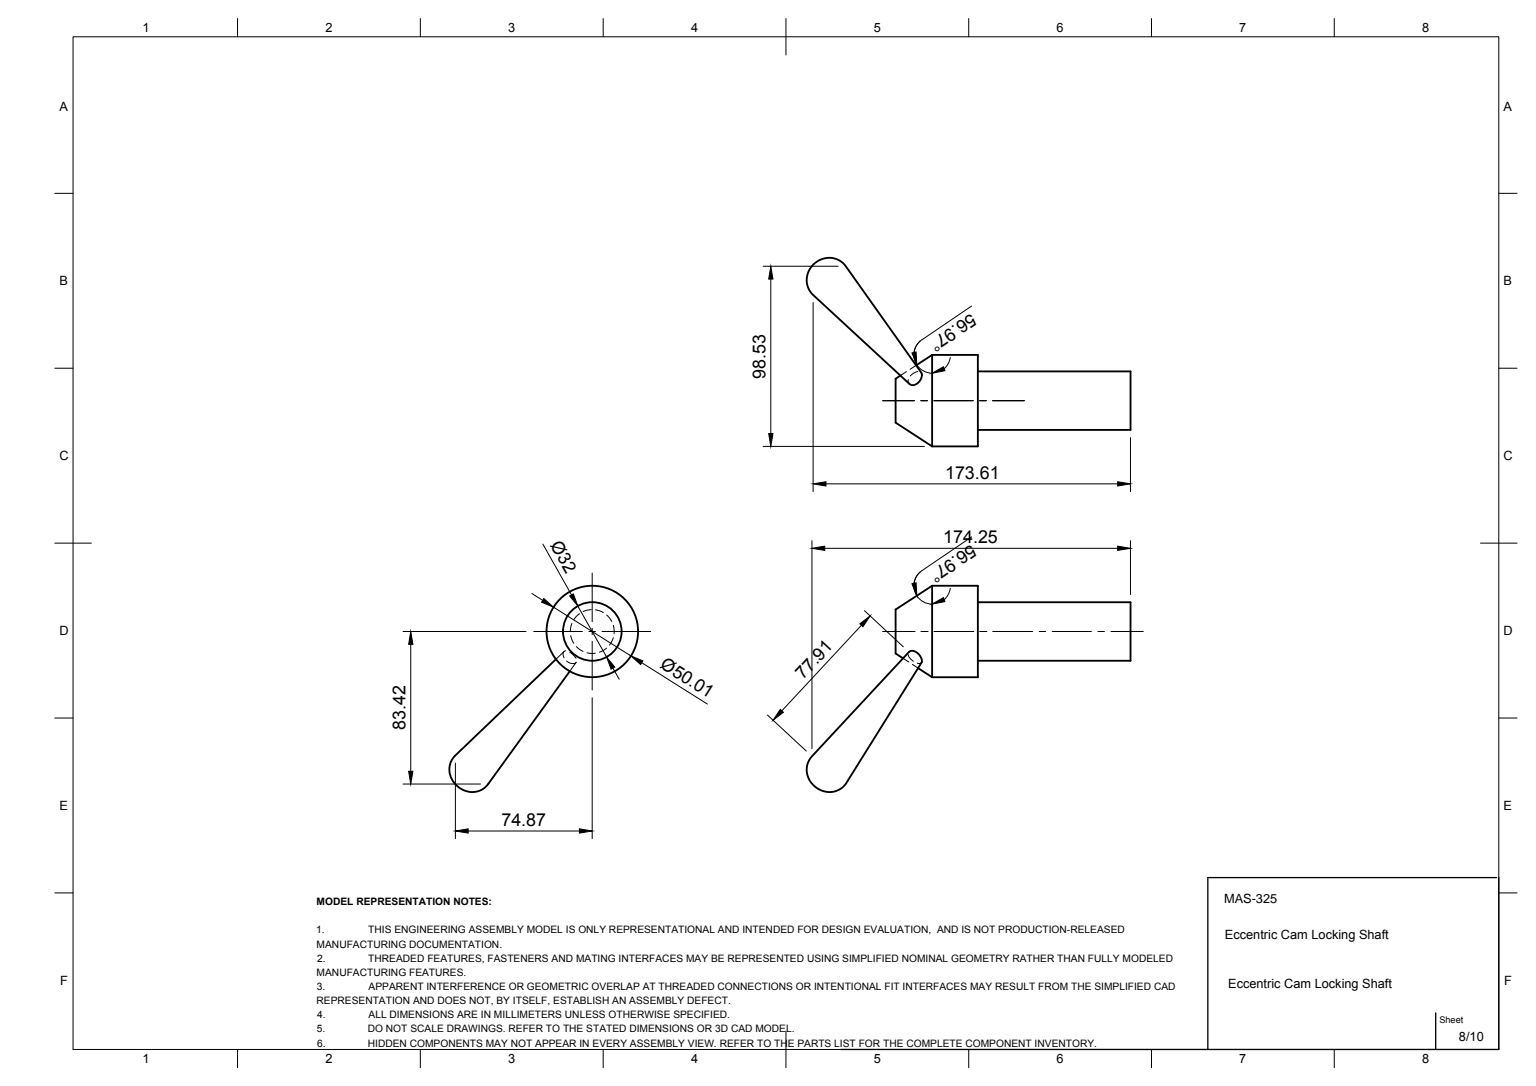
ISO-10303-21;
HEADER;
FILE_DESCRIPTION (('STEP AP214'),
    '1' );
FILE_NAME ('Eccentric Cam Locking Shaft.step',
    '2026-10-08T01:23:29',
    ( '' ),
    ( '' ),
    'SwSTEP 2.0',
    'SolidWorks 2025',
    '' );
FILE_SCHEMA (( 'AUTOMOTIVE_DESIGN' ));
ENDSEC;

DATA;
#11=CARTESIAN_POINT ( 'NONE',  ( 2.729299751253404072, 51.29764658765966345, -20.73231253916988237 ) ) ;
#218=VECTOR ( 'NONE', #39857, 1000.000000000000227 ) ;
#221=CARTESIAN_POINT ( 'NONE',  ( 0.000000000000000000, 103.6102204319011832, -100.2584055548201292 ) ) ;
#262=EDGE_CURVE ( 'NONE', #7509, #26454, #12272, .T. ) ;
#587=EDGE_CURVE ( 'NONE', #26454, #4175, #3633, .T. ) ;
#612=EDGE_CURVE ( 'NONE', #17894, #29760, #22933, .T. ) ;
#673=ORIENTED_EDGE ( 'NONE', *, *, #38806, .F. ) ;
#738=CARTESIAN_POINT ( 'NONE',  ( 0.000000000000000000, 108.6102204319011832, -108.9186595926644969 ) ) ;
#827=FACE_OUTER_BOUND ( 'NONE', #21946, .T. ) ;
#908=CARTESIAN_POINT ( 'NONE',  ( 5.761208793373444359E-16, 50.59471834446340921, -21.36672353920344491 ) ) ;
#927=DIRECTION ( 'NONE',  ( -1.000000000000000000, 0.000000000000000000, 0.000000000000000000 ) ) ;
#1275=PRODUCT_CONTEXT ( 'NONE', #38416, 'mechanical' ) ;
#1376=( GEOMETRIC_REPRESENTATION_CONTEXT ( 3 ) GLOBAL_UNCERTAINTY_ASSIGNED_CONTEXT ( ( #45358 ) ) GLOBAL_UNIT_ASSIGNED_CONTEXT ( ( #4980, #49384, #49891 ) ) REPRESENTATION_CONTEXT ( 'NONE', 'WORKASPACE' ) );
#1516=AXIS2_PLACEMENT_3D ( 'NONE', #47396, #7462, #43182 ) ;
#1542=PRESENTATION_STYLE_ASSIGNMENT (( #41212 ) ) ;
#1629=PLANE ( 'NONE',  #44758 ) ;
#1699=DIRECTION ( 'NONE',  ( 5.399917434947259359E-17, 1.000000000000000000, -0.000000000000000000 ) ) ;
#1865=DIRECTION ( 'NONE',  ( 0.000000000000000000, 0.8660254037844375974, 0.5000000000000018874 ) ) ;
#1996=EDGE_CURVE ( 'NONE', #51184, #4175, #32076, .T. ) ;
#2098=ORIENTED_EDGE ( 'NONE', *, *, #36008, .T. ) ;
#2123=AXIS2_PLACEMENT_3D ( 'NONE', #17491, #1699, #2212 ) ;
#2127=FACE_OUTER_BOUND ( 'NONE', #46157, .T. ) ;
#2180=LINE ( 'NONE', #50541, #3794 ) ;
#2212=DIRECTION ( 'NONE',  ( -1.000000000000000000, 0.000000000000000000, 0.000000000000000000 ) ) ;
#2275=CARTESIAN_POINT ( 'NONE',  ( -1.079983486989452192E-15, 45.00000000000000000, 0.000000000000000000 ) ) ;
#2365=CARTESIAN_POINT ( 'NONE',  ( -0.5864338395290236150, 50.61667155555193887, -21.34634502027464364 ) ) ;
#2916=CARTESIAN_POINT ( 'NONE',  ( 4.017037286467739499, 55.83657353238506005, -17.50344790800143358 ) ) ;
#2949=CIRCLE ( 'NONE', #2123, 25.00456841203572722 ) ;
#3096=CONICAL_SURFACE ( 'NONE', #32470, 25.00456841203573077, 0.5765357807043077765 ) ;
#3128=CARTESIAN_POINT ( 'NONE',  ( -3.363028148951364926, 51.75966409074786867, -20.33422011939856944 ) ) ;
#3176=AXIS2_PLACEMENT_3D ( 'NONE', #45599, #21409, #49549 ) ;
#3428=CARTESIAN_POINT ( 'NONE',  ( 3.372329702444478272, 56.71331670983759921, -17.05911205401795172 ) ) ;
#3572=ADVANCED_BREP_SHAPE_REPRESENTATION ( '', ( #18958, #31742 ), #42661 ) ;
#3633=CIRCLE ( 'NONE', #39709, 25.00456841203573077 ) ;
#3684=CARTESIAN_POINT ( 'NONE',  ( 1.164038952974546293, 50.70432412269159528, -21.26556842862619234 ) ) ;
#3709=FACE_OUTER_BOUND ( 'NONE', #42289, .T. ) ;
#3714=CARTESIAN_POINT ( 'NONE',  ( 0.000000000000000000, 0.000000000000000000, 0.000000000000000000 ) ) ;
#3794=VECTOR ( 'NONE', #46599, 1000.000000000000000 ) ;
#3816=ORIENTED_EDGE ( 'NONE', *, *, #6593, .F. ) ;
#3832=CARTESIAN_POINT ( 'NONE',  ( -2.429962845726266397E-15, 20.00000000000000355, 0.000000000000000000 ) ) ;
#3850=LINE ( 'NONE', #24090, #48414 ) ;
#3899=ORIENTED_EDGE ( 'NONE', *, *, #18638, .F. ) ;
#3959=CARTESIAN_POINT ( 'NONE',  ( 0.5913660303101753168, 58.11612553618076760, -16.46795210274733279 ) ) ;
#4167=VERTEX_POINT ( 'NONE', #5942 ) ;
#4175=VERTEX_POINT ( 'NONE', #21956 ) ;
#4340=ORIENTED_EDGE ( 'NONE', *, *, #33503, .T. ) ;
#4588=DIRECTION ( 'NONE',  ( 9.613575272659281827E-18, 0.4304733388468033328, -0.9026032930042329205 ) ) ;
#4657=EDGE_CURVE ( 'NONE', #4167, #4175, #43675, .T. ) ;
#4850=CIRCLE ( 'NONE', #45147, 12.00000000000000000 ) ;
#4980=( LENGTH_UNIT ( ) NAMED_UNIT ( * ) SI_UNIT ( .MILLI., .METRE. ) );
#5004=DIRECTION ( 'NONE',  ( -1.000000000000000000, 0.000000000000000000, 0.000000000000000000 ) ) ;
#5020=CARTESIAN_POINT ( 'NONE',  ( -1.600401561467127700E-24, 58.14470866581338271, -16.45750525699328293 ) ) ;
#5356=DIRECTION ( 'NONE',  ( -1.000000000000000000, 0.000000000000000000, 0.000000000000000000 ) ) ;
#5392=EDGE_LOOP ( 'NONE', ( #3816, #46775, #46312, #36724 ) ) ;
#5576=DIRECTION ( 'NONE',  ( -1.000000000000000000, 5.399917434947259359E-17, 0.000000000000000000 ) ) ;
#5647=CIRCLE ( 'NONE', #17391, 9.999999999999994671 ) ;
#5733=ORIENTED_EDGE ( 'NONE', *, *, #262, .T. ) ;
#5942=CARTESIAN_POINT ( 'NONE',  ( -25.00456841203573077, 20.00000000000000355, 0.000000000000000000 ) ) ;
#6006=FACE_OUTER_BOUND ( 'NONE', #41996, .T. ) ;
#6049=CARTESIAN_POINT ( 'NONE',  ( -1.985599386381375009, 50.94104332004447144, -21.04987985461054834 ) ) ;
#6076=( LENGTH_UNIT ( ) NAMED_UNIT ( * ) SI_UNIT ( .MILLI., .METRE. ) );
#6090=EDGE_CURVE ( 'NONE', #4175, #26454, #24966, .T. ) ;
#6175=DIRECTION ( 'NONE',  ( -1.000000000000000000, 0.000000000000000000, 0.000000000000000000 ) ) ;
#6303=CARTESIAN_POINT ( 'NONE',  ( -3.872148122484094124, 52.31912714116830898, -19.87261434340792121 ) ) ;
#6438=ORIENTED_EDGE ( 'NONE', *, *, #6090, .T. ) ;
#6468=AXIS2_PLACEMENT_3D ( 'NONE', #15552, #24728, #24217 ) ;
#6573=CARTESIAN_POINT ( 'NONE',  ( -4.232179330832529729, 52.95513942278812181, -19.37560274765787938 ) ) ;
#6593=EDGE_CURVE ( 'NONE', #34577, #29760, #32449, .T. ) ;
#7076=CARTESIAN_POINT ( 'NONE',  ( -4.008990953134272672, 52.52292218020331660, -19.70988118881478712 ) ) ;
#7097=ORIENTED_EDGE ( 'NONE', *, *, #7453, .F. ) ;
#7120=PLANE ( 'NONE',  #43869 ) ;
#7147=ORIENTED_EDGE ( 'NONE', *, *, #1996, .F. ) ;
#7354=CIRCLE ( 'NONE', #40083, 12.00000000000000000 ) ;
#7395=CARTESIAN_POINT ( 'NONE',  ( 2.248499775674169587, 57.57581846653669544, -16.67809192707658639 ) ) ;
#7453=EDGE_CURVE ( 'NONE', #48867, #44102, #9454, .T. ) ;
#7462=DIRECTION ( 'NONE',  ( -5.399917434947259359E-17, -1.000000000000000000, 0.000000000000000000 ) ) ;
#7509=VERTEX_POINT ( 'NONE', #38070 ) ;
#7637=CARTESIAN_POINT ( 'NONE',  ( -1.600401561467127700E-24, 58.14470866581338271, -16.45750525699328293 ) ) ;
#7728=AXIS2_PLACEMENT_3D ( 'NONE', #45974, #22286, #18609 ) ;
#7885=CARTESIAN_POINT ( 'NONE',  ( 4.238395535310755413, 55.36142218126918380, -17.76894564376730656 ) ) ;
#7894=ORIENTED_EDGE ( 'NONE', *, *, #7453, .T. ) ;
#7897=DIRECTION ( 'NONE',  ( 5.399917434947259359E-17, 1.000000000000000000, -0.000000000000000000 ) ) ;
#7898=DIRECTION ( 'NONE',  ( -0.5451229641719399499, -0.8383561021024406035, 6.675830932148835542E-17 ) ) ;
#8133=ORIENTED_EDGE ( 'NONE', *, *, #49350, .T. ) ;
#8189=EDGE_LOOP ( 'NONE', ( #48816, #4340, #50370, #51923 ) ) ;
#8438=DIRECTION ( 'NONE',  ( 1.000000000000000000, 0.000000000000000000, 0.000000000000000000 ) ) ;
#8536=DIRECTION ( 'NONE',  ( -1.000000000000000000, 0.000000000000000000, 0.000000000000000000 ) ) ;
#8562=ADVANCED_FACE ( 'NONE', ( #6006 ), #20320, .T. ) ;
#8670=AXIS2_PLACEMENT_3D ( 'NONE', #11175, #26427, #43236 ) ;
#8749=CYLINDRICAL_SURFACE ( 'NONE', #49830, 16.00000000000000711 ) ;
#8895=DIRECTION ( 'NONE',  ( 0.000000000000000000, 0.8660254037844375974, 0.5000000000000018874 ) ) ;
#8911=ORIENTED_EDGE ( 'NONE', *, *, #1996, .T. ) ;
#8934=LINE ( 'NONE', #24974, #21634 ) ;
#9206=CARTESIAN_POINT ( 'NONE',  ( 0.000000000000000000, 55.00653718120851465, -11.89184658936181727 ) ) ;
#9341=CARTESIAN_POINT ( 'NONE',  ( -1.079983486989452192E-15, 45.00000000000000000, 0.000000000000000000 ) ) ;
#9454=CIRCLE ( 'NONE', #18687, 16.00000000000000711 ) ;
#9497=DIRECTION ( 'NONE',  ( 5.399917434947259359E-17, 1.000000000000000000, -0.000000000000000000 ) ) ;
#9634=EDGE_LOOP ( 'NONE', ( #7097, #10302 ) ) ;
#9727=CARTESIAN_POINT ( 'NONE',  ( -1.446716803940739871, 57.92321382262407070, -16.54047372258810000 ) ) ;
#9904=ADVANCED_FACE ( 'NONE', ( #3709 ), #39962, .T. ) ;
#9997=CARTESIAN_POINT ( 'NONE',  ( -4.014990372510813366, 55.84036979173559700, -17.50138700720797402 ) ) ;
#10036=DIRECTION ( 'NONE',  ( 5.399917434947259359E-17, 1.000000000000000000, -0.000000000000000000 ) ) ;
#10060=DIRECTION ( 'NONE',  ( 0.000000000000000000, 0.8660254037844379305, 0.5000000000000012212 ) ) ;
#10256=EDGE_CURVE ( 'NONE', #17894, #39559, #5647, .T. ) ;
#10302=ORIENTED_EDGE ( 'NONE', *, *, #38879, .F. ) ;
#10539=DIRECTION ( 'NONE',  ( 1.000000000000000000, -5.399917434947259359E-17, 0.000000000000000000 ) ) ;
#10557=APPLICATION_CONTEXT ( 'automotive_design' ) ;
#10575=ORIENTED_EDGE ( 'NONE', *, *, #45851, .F. ) ;
#10576=DIRECTION ( 'NONE',  ( 5.399917434947259359E-17, 1.000000000000000000, -0.000000000000000000 ) ) ;
#10647=DIRECTION ( 'NONE',  ( 0.000000000000000000, 0.5000000000000012212, -0.8660254037844378194 ) ) ;
#10648=EDGE_CURVE ( 'NONE', #51184, #7509, #4850, .T. ) ;
#10787=EDGE_LOOP ( 'NONE', ( #30153, #13187, #43641, #23638 ) ) ;
#10819=EDGE_LOOP ( 'NONE', ( #36049, #22204 ) ) ;
#10868=EDGE_CURVE ( 'NONE', #41267, #34577, #51850, .T. ) ;
#10875=FACE_OUTER_BOUND ( 'NONE', #11864, .T. ) ;
#10901=CARTESIAN_POINT ( 'NONE',  ( 0.000000000000000000, 101.9200652401092384, -101.2342171097734536 ) ) ;
#11175=CARTESIAN_POINT ( 'NONE',  ( 0.000000000000000000, 101.5275612430648380, -100.5543802447186579 ) ) ;
#11467=CARTESIAN_POINT ( 'NONE',  ( -12.00000000000000000, 65.00000000000000000, 2.265876312981440552E-15 ) ) ;
#11499=DIRECTION ( 'NONE',  ( -1.000000000000000000, 0.000000000000000000, 0.000000000000000000 ) ) ;
#11805=AXIS2_PLACEMENT_3D ( 'NONE', #25608, #17743, #6175 ) ;
#11824=CARTESIAN_POINT ( 'NONE',  ( 4.231823864385127365, 52.95470401233406932, -19.37596056129619981 ) ) ;
#11864=EDGE_LOOP ( 'NONE', ( #7147, #3899, #5733, #13854 ) ) ;
#11901=PLANE ( 'NONE',  #44252 ) ;
#11949=PRODUCT_DEFINITION ( 'UNKNOWN', '', #45229, #43199 ) ;
#12064=DIRECTION ( 'NONE',  ( -1.000000000000000000, 0.000000000000000000, 0.000000000000000000 ) ) ;
#12272=LINE ( 'NONE', #36722, #218 ) ;
#12273=ORIENTED_EDGE ( 'NONE', *, *, #23034, .F. ) ;
#12348=ADVANCED_FACE ( 'NONE', ( #14595 ), #15055, .T. ) ;
#12817=VECTOR ( 'NONE', #4588, 1000.000000000000227 ) ;
#12941=FACE_OUTER_BOUND ( 'NONE', #13745, .T. ) ;
#12961=PRODUCT ( 'Eccentric Cam Locking Shaft', 'Eccentric Cam Locking Shaft', '', ( #1275 ) ) ;
#13066=ORIENTED_EDGE ( 'NONE', *, *, #49350, .F. ) ;
#13187=ORIENTED_EDGE ( 'NONE', *, *, #612, .F. ) ;
#13330=VECTOR ( 'NONE', #31580, 1000.000000000000000 ) ;
#13606=ORIENTED_EDGE ( 'NONE', *, *, #6593, .T. ) ;
#13738=PLANE ( 'NONE',  #32228 ) ;
#13745=EDGE_LOOP ( 'NONE', ( #20924, #49304 ) ) ;
#13854=ORIENTED_EDGE ( 'NONE', *, *, #587, .T. ) ;
#14356=ORIENTED_EDGE ( 'NONE', *, *, #33503, .F. ) ;
#14595=FACE_OUTER_BOUND ( 'NONE', #5392, .T. ) ;
#14745=ADVANCED_FACE ( 'NONE', ( #28709 ), #8749, .T. ) ;
#15055=CONICAL_SURFACE ( 'NONE', #29322, 4.042878180043863345, 0.07858164904571392217 ) ;
#15324=SHAPE_REPRESENTATION ( 'Eccentric Cam Locking Shaft', ( #31742 ), #42661 ) ;
#15459=CARTESIAN_POINT ( 'NONE',  ( 0.000000000000000000, 65.00000000000000000, 0.000000000000000000 ) ) ;
#15552=CARTESIAN_POINT ( 'NONE',  ( 0.000000000000000000, 51.50530197288473744, -13.91328567938375294 ) ) ;
#15565=CARTESIAN_POINT ( 'NONE',  ( -25.00456841203573077, 65.00000000000000000, 0.000000000000000000 ) ) ;
#16050=CARTESIAN_POINT ( 'NONE',  ( 2.246147418155142628, 51.04815051713691076, -20.95336071107404408 ) ) ;
#16823=CARTESIAN_POINT ( 'NONE',  ( 25.00456841203573077, 45.00000000000000000, 3.062176466986057355E-15 ) ) ;
#16839=LINE ( 'NONE', #9206, #19783 ) ;
#16970=FACE_OUTER_BOUND ( 'NONE', #26429, .T. ) ;
#17391=AXIS2_PLACEMENT_3D ( 'NONE', #221, #31503, #36475 ) ;
#17469=ORIENTED_EDGE ( 'NONE', *, *, #19831, .F. ) ;
#17491=CARTESIAN_POINT ( 'NONE',  ( -2.429962845726266397E-15, 20.00000000000000355, 0.000000000000000000 ) ) ;
#17743=DIRECTION ( 'NONE',  ( 5.399917434947259359E-17, 1.000000000000000000, -0.000000000000000000 ) ) ;
#17870=CLOSED_SHELL ( 'NONE', ( #8562, #9904, #21979, #22293, #26666, #41088, #49623, #34603, #27984, #22646, #14745, #12348, #46832, #51530 ) ) ;
#17894=VERTEX_POINT ( 'NONE', #19858 ) ;
#18031=CARTESIAN_POINT ( 'NONE',  ( 2.390048994689175825E-16, 100.2299100483172936, -102.2100286647267779 ) ) ;
#18113=CARTESIAN_POINT ( 'NONE',  ( -6.938893903907228378E-15, -63.50000000000000000, 0.000000000000000000 ) ) ;
#18155=DIRECTION ( 'NONE',  ( 5.399917434947259359E-17, 1.000000000000000000, -0.000000000000000000 ) ) ;
#18181=CARTESIAN_POINT ( 'NONE',  ( 0.2952580729112282976, 50.59471834446340210, -21.36672353920345202 ) ) ;
#18396=CARTESIAN_POINT ( 'NONE',  ( -2.241711803726597285, 51.04610933365329828, -20.95518423169113831 ) ) ;
#18507=ORIENTED_EDGE ( 'NONE', *, *, #34019, .T. ) ;
#18543=DIRECTION ( 'NONE',  ( -1.060575238724906545E-16, 1.000000000000000000, 0.000000000000000000 ) ) ;
#18609=DIRECTION ( 'NONE',  ( 0.000000000000000000, 0.8660254037844378194, 0.5000000000000013323 ) ) ;
#18638=EDGE_CURVE ( 'NONE', #7509, #51184, #7354, .T. ) ;
#18687=AXIS2_PLACEMENT_3D ( 'NONE', #18113, #49914, #5004 ) ;
#18693=FACE_OUTER_BOUND ( 'NONE', #10819, .T. ) ;
#18850=CARTESIAN_POINT ( 'NONE',  ( -16.00000000000001421, -63.50000000000000000, 0.000000000000000000 ) ) ;
#18945=CARTESIAN_POINT ( 'NONE',  ( 12.00000000000000000, 65.00000000000000000, 0.000000000000000000 ) ) ;
#18958=MANIFOLD_SOLID_BREP ( 'Fillet1', #17870 ) ;
#19133=EDGE_LOOP ( 'NONE', ( #13066, #43600, #18507, #21110 ) ) ;
#19165=CARTESIAN_POINT ( 'NONE',  ( -4.462159545581665832, 54.38183208324189621, -18.37010509431258498 ) ) ;
#19390=CYLINDRICAL_SURFACE ( 'NONE', #27798, 25.00456841203573077 ) ;
#19456=CARTESIAN_POINT ( 'NONE',  ( 2.958066673514105016, 57.09730180201670180, -16.88239234222090701 ) ) ;
#19713=CARTESIAN_POINT ( 'NONE',  ( 3.872902682125705542, 52.32033434345547818, -19.87165656769529321 ) ) ;
#19783=VECTOR ( 'NONE', #37046, 1000.000000000000000 ) ;
#19821=AXIS2_PLACEMENT_3D ( 'NONE', #18031, #50355, #18543 ) ;
#19831=EDGE_CURVE ( 'NONE', #39559, #47693, #21232, .T. ) ;
#19858=CARTESIAN_POINT ( 'NONE',  ( 0.000000000000000000, 111.8512453678547018, -94.59399843624255766 ) ) ;
#19983=CARTESIAN_POINT ( 'NONE',  ( 4.321872425944940588, 55.11937612772108963, -17.91061045145632846 ) ) ;
#20320=TOROIDAL_SURFACE ( 'NONE', #7728, 1.951623109906645004, 10.00000000000000000 ) ;
#20338=ORIENTED_EDGE ( 'NONE', *, *, #24629, .T. ) ;
#20917=CARTESIAN_POINT ( 'NONE',  ( -2.429962845726266397E-15, 20.00000000000000355, 0.000000000000000000 ) ) ;
#20924=ORIENTED_EDGE ( 'NONE', *, *, #19831, .T. ) ;
#21037=CARTESIAN_POINT ( 'NONE',  ( -0.2934788161349695668, 58.14470866581338271, -16.45750525699328293 ) ) ;
#21110=ORIENTED_EDGE ( 'NONE', *, *, #36008, .F. ) ;
#21232=CIRCLE ( 'NONE', #23733, 1.951623109906645226 ) ;
#21247=CARTESIAN_POINT ( 'NONE',  ( -1.600401561467127700E-24, 58.14470866581338271, -16.45750525699328293 ) ) ;
#21282=DIRECTION ( 'NONE',  ( 5.399917434947259359E-17, 1.000000000000000000, -0.000000000000000000 ) ) ;
#21409=DIRECTION ( 'NONE',  ( -0.000000000000000000, -0.5000000000000013323, 0.8660254037844380415 ) ) ;
#21634=VECTOR ( 'NONE', #21282, 1000.000000000000000 ) ;
#21836=VERTEX_POINT ( 'NONE', #28464 ) ;
#21946=EDGE_LOOP ( 'NONE', ( #14356, #20338, #26978, #40858 ) ) ;
#21956=CARTESIAN_POINT ( 'NONE',  ( -25.00456841203573077, 45.00000000000000000, 0.000000000000000000 ) ) ;
#21972=CARTESIAN_POINT ( 'NONE',  ( 16.00000000000000000, -63.50000000000000000, 1.959434878635766315E-15 ) ) ;
#21979=ADVANCED_FACE ( 'NONE', ( #38438 ), #30541, .T. ) ;
#22067=CARTESIAN_POINT ( 'NONE',  ( 5.761208793373444359E-16, 50.59471834446340921, -21.36672353920344491 ) ) ;
#22204=ORIENTED_EDGE ( 'NONE', *, *, #10648, .T. ) ;
#22286=DIRECTION ( 'NONE',  ( 0.000000000000000000, 0.5000000000000012212, -0.8660254037844378194 ) ) ;
#22292=AXIS2_PLACEMENT_3D ( 'NONE', #49190, #24742, #41281 ) ;
#22293=ADVANCED_FACE ( 'NONE', ( #16970 ), #3096, .T. ) ;
#22355=( NAMED_UNIT ( * ) PLANE_ANGLE_UNIT ( ) SI_UNIT ( $, .RADIAN. ) );
#22596=CARTESIAN_POINT ( 'NONE',  ( -4.460811323677677187, 53.88842563715992640, -18.70041964591998607 ) ) ;
#22646=ADVANCED_FACE ( 'NONE', ( #24265 ), #11901, .F. ) ;
#22933=CIRCLE ( 'NONE', #8670, 11.92076361695220932 ) ;
#23034=EDGE_CURVE ( 'NONE', #29760, #17894, #25832, .T. ) ;
#23418=CARTESIAN_POINT ( 'NONE',  ( 0.2934699642939896380, 58.14470866581339692, -16.45750525699327937 ) ) ;
#23426=AXIS2_PLACEMENT_3D ( 'NONE', #20917, #36937, #927 ) ;
#23638=ORIENTED_EDGE ( 'NONE', *, *, #44973, .F. ) ;
#23733=AXIS2_PLACEMENT_3D ( 'NONE', #41540, #25519, #1865 ) ;
#23914=CARTESIAN_POINT ( 'NONE',  ( 3.555982085019433914, 56.50744240459307832, -17.15800186250228876 ) ) ;
#23927=DIRECTION ( 'NONE',  ( -1.000000000000000000, 0.000000000000000000, 0.000000000000000000 ) ) ;
#24090=CARTESIAN_POINT ( 'NONE',  ( 25.00456841203573077, 65.00000000000000000, 3.062176466986057355E-15 ) ) ;
#24107=AXIS2_PLACEMENT_3D ( 'NONE', #35731, #31529, #12064 ) ;
#24217=DIRECTION ( 'NONE',  ( 0.000000000000000000, 0.8660254037844379305, 0.5000000000000011102 ) ) ;
#24265=FACE_OUTER_BOUND ( 'NONE', #9634, .T. ) ;
#24425=AXIS2_PLACEMENT_3D ( 'NONE', #3832, #51939, #8536 ) ;
#24629=EDGE_CURVE ( 'NONE', #44745, #4167, #2949, .T. ) ;
#24728=DIRECTION ( 'NONE',  ( 0.000000000000000000, 0.5000000000000012212, -0.8660254037844378194 ) ) ;
#24742=DIRECTION ( 'NONE',  ( 5.399917434947259359E-17, 1.000000000000000000, -0.000000000000000000 ) ) ;
#24789=CARTESIAN_POINT ( 'NONE',  ( 0.000000000000000000, 65.00000000000000000, 0.000000000000000000 ) ) ;
#24840=DIRECTION ( 'NONE',  ( 1.000000000000000000, 0.000000000000000000, 0.000000000000000000 ) ) ;
#24947=EDGE_CURVE ( 'NONE', #41267, #17894, #16839, .T. ) ;
#24966=CIRCLE ( 'NONE', #24107, 25.00456841203573077 ) ;
#24974=CARTESIAN_POINT ( 'NONE',  ( -16.00000000000000711, 65.00000000000000000, 0.000000000000000000 ) ) ;
#25321=EDGE_CURVE ( 'NONE', #29760, #47693, #42482, .T. ) ;
#25382=CIRCLE ( 'NONE', #32081, 1.951623109906645226 ) ;
#25519=DIRECTION ( 'NONE',  ( 0.000000000000000000, 0.5000000000000013323, -0.8660254037844380415 ) ) ;
#25555=CARTESIAN_POINT ( 'NONE',  ( 0.000000000000000000, 95.86090687668166765, -116.2794792057534607 ) ) ;
#25608=CARTESIAN_POINT ( 'NONE',  ( -6.938893903907228378E-15, -63.50000000000000000, 0.000000000000000000 ) ) ;
#25758=CARTESIAN_POINT ( 'NONE',  ( -1.985634459154583364, 57.70970895460362726, -16.62426742705180871 ) ) ;
#25832=CIRCLE ( 'NONE', #3176, 11.92076361695220932 ) ;
#26012=CARTESIAN_POINT ( 'NONE',  ( -2.954493006721953030, 51.44106513229385769, -20.60687412731818213 ) ) ;
#26427=DIRECTION ( 'NONE',  ( -0.000000000000000000, -0.5000000000000013323, 0.8660254037844380415 ) ) ;
#26429=EDGE_LOOP ( 'NONE', ( #48434, #8911, #6438, #42213 ) ) ;
#26454=VERTEX_POINT ( 'NONE', #16823 ) ;
#26516=CARTESIAN_POINT ( 'NONE',  ( -3.547000324993504261, 51.93490815224947710, -20.18691131683817730 ) ) ;
#26666=ADVANCED_FACE ( 'NONE', ( #39355 ), #19390, .T. ) ;
#26920=DIRECTION ( 'NONE',  ( 0.000000000000000000, 0.5000000000000012212, -0.8660254037844378194 ) ) ;
#26978=ORIENTED_EDGE ( 'NONE', *, *, #4657, .T. ) ;
#27030=CARTESIAN_POINT ( 'NONE',  ( -4.322350346021930356, 55.11748258468679751, -17.91176154419416378 ) ) ;
#27079=CARTESIAN_POINT ( 'NONE',  ( 3.366759895602029928, 51.76293813683449230, -20.33144901513888314 ) ) ;
#27150=FACE_BOUND ( 'NONE', #51512, .T. ) ;
#27309=CARTESIAN_POINT ( 'NONE',  ( 25.00456841203572367, 20.00000000000000355, 3.062176466986057355E-15 ) ) ;
#27622=CARTESIAN_POINT ( 'NONE',  ( 3.499092996509686644E-32, 65.00000000000000000, 0.000000000000000000 ) ) ;
#27798=AXIS2_PLACEMENT_3D ( 'NONE', #15459, #31466, #11499 ) ;
#27853=CARTESIAN_POINT ( 'NONE',  ( 4.316855663795568177, 53.18022804202947640, -19.20662862702307194 ) ) ;
#27984=ADVANCED_FACE ( 'NONE', ( #18693 ), #7120, .F. ) ;
#28118=CARTESIAN_POINT ( 'NONE',  ( -25.00456841203573077, 45.00000000000000000, 3.062176466986057355E-15 ) ) ;
#28464=CARTESIAN_POINT ( 'NONE',  ( -16.00000000000000711, 20.00000000000000355, 0.000000000000000000 ) ) ;
#28709=FACE_OUTER_BOUND ( 'NONE', #19133, .T. ) ;
#29028=DIRECTION ( 'NONE',  ( -5.399917434947259359E-17, -1.000000000000000000, 0.000000000000000000 ) ) ;
#29322=AXIS2_PLACEMENT_3D ( 'NONE', #42713, #10647, #34799 ) ;
#29647=CIRCLE ( 'NONE', #49813, 25.00456841203572722 ) ;
#29760=VERTEX_POINT ( 'NONE', #36372 ) ;
#30153=ORIENTED_EDGE ( 'NONE', *, *, #25321, .F. ) ;
#30463=CARTESIAN_POINT ( 'NONE',  ( -0.2952669786863603152, 50.59471834446340921, -21.36672353920344847 ) ) ;
#30541=CYLINDRICAL_SURFACE ( 'NONE', #44208, 16.00000000000000711 ) ;
#30595=FACE_OUTER_BOUND ( 'NONE', #10787, .T. ) ;
#30606=EDGE_LOOP ( 'NONE', ( #7894, #8133, #673, #35363 ) ) ;
#30620=ORIENTED_EDGE ( 'NONE', *, *, #37871, .F. ) ;
#30714=CARTESIAN_POINT ( 'NONE',  ( -3.556303009769684831, 56.50711438170559120, -17.15815478421502505 ) ) ;
#31285=CARTESIAN_POINT ( 'NONE',  ( 1.445069716139520066, 57.92390192091106371, -16.54020211540079899 ) ) ;
#31363=DIRECTION ( 'NONE',  ( 5.399917434947259359E-17, 1.000000000000000000, -0.000000000000000000 ) ) ;
#31466=DIRECTION ( 'NONE',  ( 5.399917434947259359E-17, 1.000000000000000000, -0.000000000000000000 ) ) ;
#31503=DIRECTION ( 'NONE',  ( -1.000000000000000000, 0.000000000000000000, 0.000000000000000000 ) ) ;
#31529=DIRECTION ( 'NONE',  ( 5.399917434947259359E-17, 1.000000000000000000, -0.000000000000000000 ) ) ;
#31580=DIRECTION ( 'NONE',  ( 5.399917434947259359E-17, 1.000000000000000000, -0.000000000000000000 ) ) ;
#31742=AXIS2_PLACEMENT_3D ( 'NONE', #3714, #31843, #8438 ) ;
#31816=CARTESIAN_POINT ( 'NONE',  ( 2.957638829135800673, 51.44316066764527307, -20.60505050678383654 ) ) ;
#31843=DIRECTION ( 'NONE',  ( 0.000000000000000000, 0.000000000000000000, 1.000000000000000000 ) ) ;
#32058=CARTESIAN_POINT ( 'NONE',  ( 4.434257923028284587, 54.62691647646887816, -18.21285284460631360 ) ) ;
#32076=LINE ( 'NONE', #28118, #48469 ) ;
#32081=AXIS2_PLACEMENT_3D ( 'NONE', #37787, #37539, #8895 ) ;
#32228=AXIS2_PLACEMENT_3D ( 'NONE', #25555, #46076, #10060 ) ;
#32254=EDGE_LOOP ( 'NONE', ( #43657, #2098 ) ) ;
#32393=DIRECTION ( 'NONE',  ( -1.000000000000000000, 5.399917434947259359E-17, 0.000000000000000000 ) ) ;
#32449=LINE ( 'NONE', #48499, #12817 ) ;
#32470=AXIS2_PLACEMENT_3D ( 'NONE', #9341, #29028, #24840 ) ;
#33141=CYLINDRICAL_SURFACE ( 'NONE', #22292, 25.00456841203573077 ) ;
#33421=CONICAL_SURFACE ( 'NONE', #1516, 25.00456841203573077, 0.5765357807043077765 ) ;
#33424=DIRECTION ( 'NONE',  ( -1.000000000000000000, 0.000000000000000000, 0.000000000000000000 ) ) ;
#33503=EDGE_CURVE ( 'NONE', #44745, #26454, #3850, .T. ) ;
#33770=UNCERTAINTY_MEASURE_WITH_UNIT (LENGTH_MEASURE( 1.000000000000000082E-05 ), #6076, 'distance_accuracy_value', 'NONE');
#33851=FILL_AREA_STYLE ('',( #45695 ) ) ;
#33889=CARTESIAN_POINT ( 'NONE',  ( -1.162868876050039635, 58.00636336259468351, -16.50905505121457750 ) ) ;
#33925=FACE_BOUND ( 'NONE', #32254, .T. ) ;
#34019=EDGE_CURVE ( 'NONE', #48867, #21836, #8934, .T. ) ;
#34155=CARTESIAN_POINT ( 'NONE',  ( -3.368532359847667301, 56.71706743982079502, -17.05735933465977894 ) ) ;
#34208=CARTESIAN_POINT ( 'NONE',  ( 0.5906848879318955525, 50.61712177749316055, -21.34592841102499250 ) ) ;
#34577=VERTEX_POINT ( 'NONE', #50832 ) ;
#34603=ADVANCED_FACE ( 'NONE', ( #10875, #27150 ), #33421, .T. ) ;
#34799=DIRECTION ( 'NONE',  ( 0.000000000000000000, 0.8660254037844379305, 0.5000000000000011102 ) ) ;
#35229=CARTESIAN_POINT ( 'NONE',  ( 1.988269209400828741, 57.70862950595167007, -16.62469262932894409 ) ) ;
#35309=CARTESIAN_POINT ( 'NONE',  ( 16.00000000000000000, 20.00000000000000355, 1.959434878635766315E-15 ) ) ;
#35363=ORIENTED_EDGE ( 'NONE', *, *, #34019, .F. ) ;
#35480=CARTESIAN_POINT ( 'NONE',  ( 2.731537303769431269, 57.27118962484799169, -16.80650863900784131 ) ) ;
#35731=CARTESIAN_POINT ( 'NONE',  ( -1.079983486989452192E-15, 45.00000000000000000, 0.000000000000000000 ) ) ;
#35743=CARTESIAN_POINT ( 'NONE',  ( 4.431967298689001744, 53.65124805090443516, -18.86592383872149981 ) ) ;
#36008=EDGE_CURVE ( 'NONE', #40165, #21836, #46103, .T. ) ;
#36049=ORIENTED_EDGE ( 'NONE', *, *, #18638, .T. ) ;
#36338=CARTESIAN_POINT ( 'NONE',  ( -6.938893903907228378E-15, -63.50000000000000000, 0.000000000000000000 ) ) ;
#36372=CARTESIAN_POINT ( 'NONE',  ( 1.459872500689274649E-15, 91.20387711827495991, -106.5147620531948007 ) ) ;
#36475=DIRECTION ( 'NONE',  ( 0.000000000000000000, 0.000000000000000000, 1.000000000000000000 ) ) ;
#36722=CARTESIAN_POINT ( 'NONE',  ( 25.00456841203573077, 45.00000000000000000, 0.000000000000000000 ) ) ;
#36724=ORIENTED_EDGE ( 'NONE', *, *, #612, .T. ) ;
#36753=CARTESIAN_POINT ( 'NONE',  ( 2.390048994689182728E-16, 105.2299100483173078, -110.8702827025711599 ) ) ;
#36880=DIRECTION ( 'NONE',  ( -1.000000000000000000, 0.000000000000000000, 0.000000000000000000 ) ) ;
#36937=DIRECTION ( 'NONE',  ( 5.399917434947259359E-17, 1.000000000000000000, -0.000000000000000000 ) ) ;
#37046=DIRECTION ( 'NONE',  ( 0.000000000000000000, 0.5664407118577555744, -0.8241024935953531472 ) ) ;
#37056=CARTESIAN_POINT ( 'NONE',  ( -0.5847574683125812411, 58.11708756977395041, -16.46759551110862674 ) ) ;
#37539=DIRECTION ( 'NONE',  ( 0.000000000000000000, 0.5000000000000013323, -0.8660254037844380415 ) ) ;
#37617=CARTESIAN_POINT ( 'NONE',  ( -2.429962845726266397E-15, 20.00000000000000355, 0.000000000000000000 ) ) ;
#37787=CARTESIAN_POINT ( 'NONE',  ( 0.000000000000000000, 106.9200652401092526, -109.8944711476178213 ) ) ;
#37871=EDGE_CURVE ( 'NONE', #34577, #41267, #44015, .T. ) ;
#38070=CARTESIAN_POINT ( 'NONE',  ( 12.00000000000000000, 65.00000000000000000, 0.000000000000000000 ) ) ;
#38279=COLOUR_RGB ( '', 0.72549020, 0.75294118, 0.79215686) ;
#38416=APPLICATION_CONTEXT ( 'automotive_design' ) ;
#38438=FACE_OUTER_BOUND ( 'NONE', #30606, .T. ) ;
#38609=CARTESIAN_POINT ( 'NONE',  ( -2.733443440668967384, 57.27004613166161562, -16.80698578740291538 ) ) ;
#38806=EDGE_CURVE ( 'NONE', #21836, #40165, #51293, .T. ) ;
#38879=EDGE_CURVE ( 'NONE', #44102, #48867, #42875, .T. ) ;
#39116=CARTESIAN_POINT ( 'NONE',  ( -4.431386850739163386, 53.64904251590335349, -18.86752773431649999 ) ) ;
#39175=CARTESIAN_POINT ( 'NONE',  ( 4.010723116466015092, 52.52602521353311005, -19.70746035629181847 ) ) ;
#39355=FACE_OUTER_BOUND ( 'NONE', #8189, .T. ) ;
#39499=ORIENTED_EDGE ( 'NONE', *, *, #10256, .F. ) ;
#39559=VERTEX_POINT ( 'NONE', #738 ) ;
#39671=CARTESIAN_POINT ( 'NONE',  ( 4.460702607355470306, 53.89045795899486535, -18.69908610442183772 ) ) ;
#39709=AXIS2_PLACEMENT_3D ( 'NONE', #2275, #47199, #42196 ) ;
#39813=ORIENTED_EDGE ( 'NONE', *, *, #25321, .T. ) ;
#39857=DIRECTION ( 'NONE',  ( 0.5451229641719399499, -0.8383561021024406035, 0.000000000000000000 ) ) ;
#39931=CARTESIAN_POINT ( 'NONE',  ( 1.165667945738152245, 58.00551856110927673, -16.50937507019845540 ) ) ;
#39962=CONICAL_SURFACE ( 'NONE', #6468, 4.042878180043863345, 0.07858164904571392217 ) ;
#40083=AXIS2_PLACEMENT_3D ( 'NONE', #46282, #18155, #45752 ) ;
#40165=VERTEX_POINT ( 'NONE', #35309 ) ;
#40803=DIRECTION ( 'NONE',  ( 5.399917434947259359E-17, 1.000000000000000000, -0.000000000000000000 ) ) ;
#40858=ORIENTED_EDGE ( 'NONE', *, *, #587, .F. ) ;
#41088=ADVANCED_FACE ( 'NONE', ( #2127, #33925 ), #1629, .F. ) ;
#41212=SURFACE_STYLE_USAGE ( .BOTH. , #41470 ) ;
#41267=VERTEX_POINT ( 'NONE', #21247 ) ;
#41281=DIRECTION ( 'NONE',  ( -1.000000000000000000, 0.000000000000000000, 0.000000000000000000 ) ) ;
#41470=SURFACE_SIDE_STYLE ('',( #41746 ) ) ;
#41540=CARTESIAN_POINT ( 'NONE',  ( 0.000000000000000000, 106.9200652401092526, -109.8944711476178213 ) ) ;
#41746=SURFACE_STYLE_FILL_AREA ( #33851 ) ;
#41792=CARTESIAN_POINT ( 'NONE',  ( -2.245234434168357218, 57.57781898212405025, -16.67725351333963602 ) ) ;
#41996=EDGE_LOOP ( 'NONE', ( #12273, #39813, #17469, #39499 ) ) ;
#42036=CARTESIAN_POINT ( 'NONE',  ( -3.878716889882891650, 56.06915626585696089, -17.38004533314371969 ) ) ;
#42196=DIRECTION ( 'NONE',  ( -1.000000000000000000, 0.000000000000000000, 0.000000000000000000 ) ) ;
#42213=ORIENTED_EDGE ( 'NONE', *, *, #262, .F. ) ;
#42289=EDGE_LOOP ( 'NONE', ( #30620, #13606, #44977, #45893 ) ) ;
#42482=CIRCLE ( 'NONE', #19821, 9.999999999999994671 ) ;
#42484=STYLED_ITEM ( 'NONE', ( #1542 ), #18958 ) ;
#42552=CARTESIAN_POINT ( 'NONE',  ( -4.317676980897452665, 53.18341953714510595, -19.20431157105264219 ) ) ;
#42661=( GEOMETRIC_REPRESENTATION_CONTEXT ( 3 ) GLOBAL_UNCERTAINTY_ASSIGNED_CONTEXT ( ( #33770 ) ) GLOBAL_UNIT_ASSIGNED_CONTEXT ( ( #6076, #22355, #46288 ) ) REPRESENTATION_CONTEXT ( 'NONE', 'WORKASPACE' ) );
#42713=CARTESIAN_POINT ( 'NONE',  ( 0.000000000000000000, 51.50530197288473744, -13.91328567938375294 ) ) ;
#42875=CIRCLE ( 'NONE', #11805, 16.00000000000000711 ) ;
#43182=DIRECTION ( 'NONE',  ( 1.000000000000000000, 0.000000000000000000, 0.000000000000000000 ) ) ;
#43199=PRODUCT_DEFINITION_CONTEXT ( 'detailed design', #10557, 'design' ) ;
#43236=DIRECTION ( 'NONE',  ( 0.000000000000000000, -0.8660254037844378194, -0.5000000000000012212 ) ) ;
#43388=CARTESIAN_POINT ( 'NONE',  ( 1.989912926925674563, 50.94255943192818137, -21.04850772462241082 ) ) ;
#43442=MECHANICAL_DESIGN_GEOMETRIC_PRESENTATION_REPRESENTATION('',(#42484),#1376);
#43600=ORIENTED_EDGE ( 'NONE', *, *, #38879, .T. ) ;
#43638=CARTESIAN_POINT ( 'NONE',  ( 1.446991361456883896, 50.76983389525828727, -21.20535062037070517 ) ) ;
#43641=ORIENTED_EDGE ( 'NONE', *, *, #10256, .T. ) ;
#43657=ORIENTED_EDGE ( 'NONE', *, *, #38806, .T. ) ;
#43675=LINE ( 'NONE', #15565, #13330 ) ;
#43869=AXIS2_PLACEMENT_3D ( 'NONE', #18945, #46554, #10539 ) ;
#43890=CARTESIAN_POINT ( 'NONE',  ( 3.877854670627010947, 56.07043499712327872, -17.37938424498008771 ) ) ;
#44015=B_SPLINE_CURVE_WITH_KNOTS ( 'NONE', 3,
 ( #908, #18181, #34208, #3684, #43638, #43388, #16050, #11, #31816, #27079, #47075, #19713, #39175, #11824, #27853, #35743, #39671, #47854, #32058, #19983, #7885, #2916, #43890, #23914, #3428, #19456, #35480, #7395, #35229, #31285, #39931, #3959, #23418, #7637 ),
 .UNSPECIFIED., .F., .F.,
 ( 4, 2, 2, 2, 2, 2, 2, 2, 2, 2, 2, 2, 2, 2, 2, 2, 4 ),
 ( 0.004374701946809896047, 0.005252622471382774154, 0.006130542995955652261, 0.007008463520528530367, 0.007886384045101408474, 0.008764304569674287448, 0.009642225094247164688, 0.01052014561882004193, 0.01139806614339292090, 0.01227598666796579988, 0.01315390719253867712, 0.01403182771711155435, 0.01490974824168443333, 0.01578766876625731230, 0.01666558929083018781, 0.01754350981540306678, 0.01842143033997594576 ),
 .UNSPECIFIED. ) ;
#44102=VERTEX_POINT ( 'NONE', #21972 ) ;
#44208=AXIS2_PLACEMENT_3D ( 'NONE', #46593, #10576, #5356 ) ;
#44252=AXIS2_PLACEMENT_3D ( 'NONE', #36338, #31363, #32393 ) ;
#44745=VERTEX_POINT ( 'NONE', #27309 ) ;
#44758=AXIS2_PLACEMENT_3D ( 'NONE', #49975, #10036, #5576 ) ;
#44973=EDGE_CURVE ( 'NONE', #47693, #39559, #25382, .T. ) ;
#44977=ORIENTED_EDGE ( 'NONE', *, *, #23034, .T. ) ;
#45147=AXIS2_PLACEMENT_3D ( 'NONE', #27622, #7897, #23927 ) ;
#45195=SHAPE_DEFINITION_REPRESENTATION ( #50371, #15324 ) ;
#45229=PRODUCT_DEFINITION_FORMATION_WITH_SPECIFIED_SOURCE ( 'ANY', '', #12961, .NOT_KNOWN. ) ;
#45358=UNCERTAINTY_MEASURE_WITH_UNIT (LENGTH_MEASURE( 1.000000000000000082E-05 ), #4980, 'distance_accuracy_value', 'NONE');
#45584=ORIENTED_EDGE ( 'NONE', *, *, #37871, .T. ) ;
#45599=CARTESIAN_POINT ( 'NONE',  ( 0.000000000000000000, 101.5275612430648380, -100.5543802447186579 ) ) ;
#45695=FILL_AREA_STYLE_COLOUR ( '', #38279 ) ;
#45752=DIRECTION ( 'NONE',  ( -1.000000000000000000, 0.000000000000000000, 0.000000000000000000 ) ) ;
#45851=EDGE_CURVE ( 'NONE', #4167, #44745, #29647, .T. ) ;
#45893=ORIENTED_EDGE ( 'NONE', *, *, #24947, .F. ) ;
#45974=CARTESIAN_POINT ( 'NONE',  ( 0.000000000000000000, 101.9200652401092384, -101.2342171097734536 ) ) ;
#46010=CARTESIAN_POINT ( 'NONE',  ( -4.237343245523132573, 55.36427016545908231, -17.76729481263095067 ) ) ;
#46076=DIRECTION ( 'NONE',  ( 0.000000000000000000, 0.5000000000000012212, -0.8660254037844379305 ) ) ;
#46103=CIRCLE ( 'NONE', #23426, 16.00000000000000355 ) ;
#46157=EDGE_LOOP ( 'NONE', ( #10575, #48256 ) ) ;
#46282=CARTESIAN_POINT ( 'NONE',  ( 3.499092996509686644E-32, 65.00000000000000000, 0.000000000000000000 ) ) ;
#46288=( NAMED_UNIT ( * ) SI_UNIT ( $, .STERADIAN. ) SOLID_ANGLE_UNIT ( ) );
#46312=ORIENTED_EDGE ( 'NONE', *, *, #24947, .T. ) ;
#46393=DIRECTION ( 'NONE',  ( 0.000000000000000000, 0.8660254037844378194, 0.5000000000000013323 ) ) ;
#46554=DIRECTION ( 'NONE',  ( -5.399917434947259359E-17, -1.000000000000000000, 0.000000000000000000 ) ) ;
#46593=CARTESIAN_POINT ( 'NONE',  ( 0.000000000000000000, 65.00000000000000000, 0.000000000000000000 ) ) ;
#46599=DIRECTION ( 'NONE',  ( 5.399917434947259359E-17, 1.000000000000000000, -0.000000000000000000 ) ) ;
#46775=ORIENTED_EDGE ( 'NONE', *, *, #10868, .F. ) ;
#46832=ADVANCED_FACE ( 'NONE', ( #12941 ), #13738, .T. ) ;
#47026=CARTESIAN_POINT ( 'NONE',  ( -2.727113817024051201, 51.29627183467966489, -20.73351566952182878 ) ) ;
#47075=CARTESIAN_POINT ( 'NONE',  ( 3.549863570076594588, 51.93797953136993328, -20.18436947879331456 ) ) ;
#47199=DIRECTION ( 'NONE',  ( 5.399917434947259359E-17, 1.000000000000000000, -0.000000000000000000 ) ) ;
#47396=CARTESIAN_POINT ( 'NONE',  ( -1.079983486989452192E-15, 45.00000000000000000, 0.000000000000000000 ) ) ;
#47693=VERTEX_POINT ( 'NONE', #36753 ) ;
#47854=CARTESIAN_POINT ( 'NONE',  ( 4.462259530680975139, 54.37685667866154660, -18.37340906701131615 ) ) ;
#48256=ORIENTED_EDGE ( 'NONE', *, *, #24629, .F. ) ;
#48414=VECTOR ( 'NONE', #51957, 1000.000000000000000 ) ;
#48434=ORIENTED_EDGE ( 'NONE', *, *, #10648, .F. ) ;
#48469=VECTOR ( 'NONE', #7898, 1000.000000000000227 ) ;
#48499=CARTESIAN_POINT ( 'NONE',  ( 4.951097822533392803E-16, 48.00406676456095312, -15.93472476940568860 ) ) ;
#48816=ORIENTED_EDGE ( 'NONE', *, *, #45851, .T. ) ;
#48867=VERTEX_POINT ( 'NONE', #18850 ) ;
#49180=ORIENTED_EDGE ( 'NONE', *, *, #10868, .T. ) ;
#49190=CARTESIAN_POINT ( 'NONE',  ( 0.000000000000000000, 65.00000000000000000, 0.000000000000000000 ) ) ;
#49304=ORIENTED_EDGE ( 'NONE', *, *, #44973, .T. ) ;
#49350=EDGE_CURVE ( 'NONE', #44102, #40165, #2180, .T. ) ;
#49384=( NAMED_UNIT ( * ) PLANE_ANGLE_UNIT ( ) SI_UNIT ( $, .RADIAN. ) );
#49549=DIRECTION ( 'NONE',  ( 0.000000000000000000, -0.8660254037844378194, -0.5000000000000012212 ) ) ;
#49623=ADVANCED_FACE ( 'NONE', ( #827 ), #33141, .T. ) ;
#49813=AXIS2_PLACEMENT_3D ( 'NONE', #37617, #9497, #33424 ) ;
#49830=AXIS2_PLACEMENT_3D ( 'NONE', #24789, #40803, #36880 ) ;
#49891=( NAMED_UNIT ( * ) SI_UNIT ( $, .STERADIAN. ) SOLID_ANGLE_UNIT ( ) );
#49914=DIRECTION ( 'NONE',  ( 5.399917434947259359E-17, 1.000000000000000000, -0.000000000000000000 ) ) ;
#49935=CARTESIAN_POINT ( 'NONE',  ( -1.446433552754633256, 50.76980153716073829, -21.20538461533670116 ) ) ;
#49975=CARTESIAN_POINT ( 'NONE',  ( 16.00000000000000000, 20.00000000000000355, 0.000000000000000000 ) ) ;
#50187=AXIS2_PLACEMENT_3D ( 'NONE', #10901, #26920, #46393 ) ;
#50207=CARTESIAN_POINT ( 'NONE',  ( -1.160780020586678285, 50.70363469020618652, -21.26620207273386498 ) ) ;
#50355=DIRECTION ( 'NONE',  ( 1.000000000000000000, 1.060575238724905929E-16, 6.123233995736780827E-17 ) ) ;
#50370=ORIENTED_EDGE ( 'NONE', *, *, #6090, .F. ) ;
#50371=PRODUCT_DEFINITION_SHAPE ( 'NONE', 'NONE',  #11949 ) ;
#50485=SHAPE_REPRESENTATION_RELATIONSHIP ( 'NONE' , 'NONE' ,  #15324, #3572 ) ;
#50541=CARTESIAN_POINT ( 'NONE',  ( 16.00000000000000711, 65.00000000000000000, 1.959434878635766315E-15 ) ) ;
#50710=CARTESIAN_POINT ( 'NONE',  ( -2.957822182692360080, 57.09729520864777896, -16.88242217723719918 ) ) ;
#50832=CARTESIAN_POINT ( 'NONE',  ( 5.761208793373444359E-16, 50.59471834446340921, -21.36672353920344491 ) ) ;
#50976=CARTESIAN_POINT ( 'NONE',  ( -4.434052336286734786, 54.62761619819747949, -18.21243447522283532 ) ) ;
#51013=TOROIDAL_SURFACE ( 'NONE', #50187, 1.951623109906645004, 10.00000000000000000 ) ;
#51184=VERTEX_POINT ( 'NONE', #11467 ) ;
#51293=CIRCLE ( 'NONE', #24425, 16.00000000000000355 ) ;
#51512=EDGE_LOOP ( 'NONE', ( #49180, #45584 ) ) ;
#51530=ADVANCED_FACE ( 'NONE', ( #30595 ), #51013, .T. ) ;
#51850=B_SPLINE_CURVE_WITH_KNOTS ( 'NONE', 3,
 ( #5020, #21037, #37056, #33889, #9727, #25758, #41792, #38609, #50710, #34155, #30714, #42036, #9997, #46010, #27030, #50976, #19165, #22596, #39116, #42552, #6573, #7076, #6303, #26516, #3128, #26012, #47026, #18396, #6049, #49935, #50207, #2365, #30463, #22067 ),
 .UNSPECIFIED., .F., .F.,
 ( 4, 2, 2, 2, 2, 2, 2, 2, 2, 2, 2, 2, 2, 2, 2, 2, 4 ),
 ( 0.01842143033997594576, 0.01929937734498573393, 0.02017732434999552210, 0.02105527135500531027, 0.02193321836001509845, 0.02281116536502488315, 0.02368911237003466785, 0.02456705937504445950, 0.02544500638005424420, 0.02632295338506403237, 0.02720090039007382055, 0.02807884739508360872, 0.02895679440009339689, 0.02983474140510318506, 0.03071268841011297324, 0.03159063541512276141, 0.03246858242013254958 ),
 .UNSPECIFIED. ) ;
#51923=ORIENTED_EDGE ( 'NONE', *, *, #4657, .F. ) ;
#51939=DIRECTION ( 'NONE',  ( 5.399917434947259359E-17, 1.000000000000000000, -0.000000000000000000 ) ) ;
#51957=DIRECTION ( 'NONE',  ( 5.399917434947259359E-17, 1.000000000000000000, -0.000000000000000000 ) ) ;
ENDSEC;
END-ISO-10303-21;
